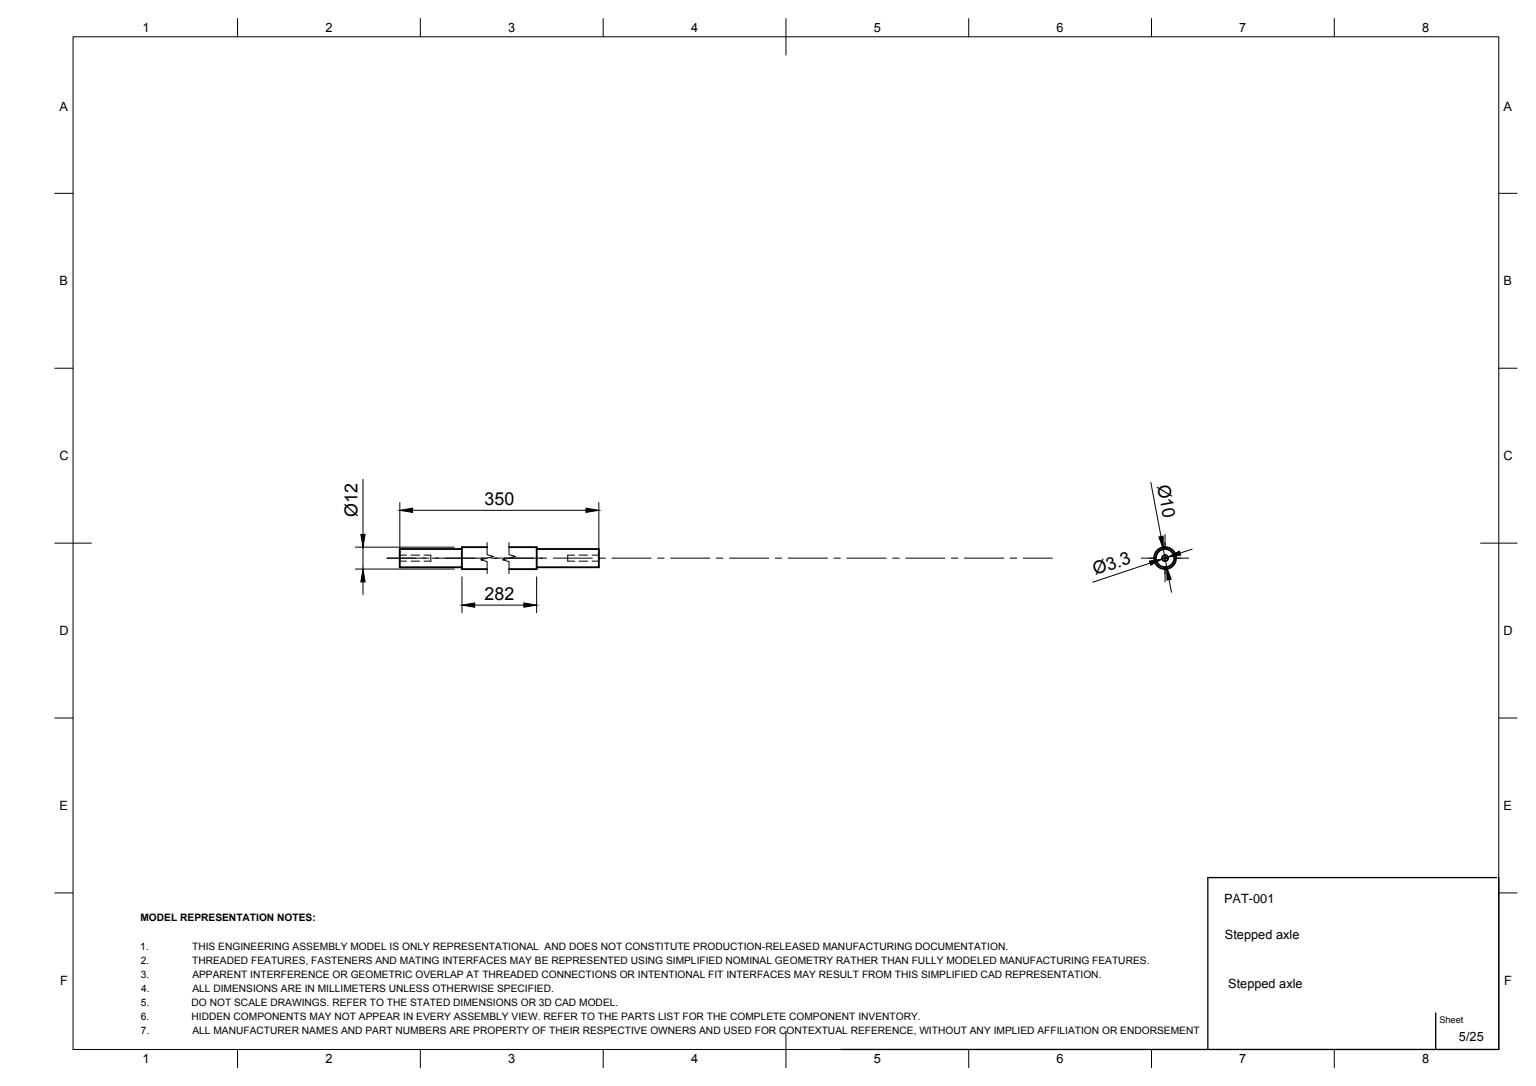
ISO-10303-21;
HEADER;
/* Generated by software containing ST-Developer
 * from STEP Tools, Inc. (www.steptools.com) 
 */

FILE_DESCRIPTION(
/* description */ ('PAT-001'),
/* implementation_level */ '2;1');

FILE_NAME(
/* name */ 'Stepped axle.step',
/* time_stamp */ '2026-10-29T17:07:15-07:00',
/* author */ (''),
/* organization */ (''),
/* preprocessor_version */ 'ST-DEVELOPER v20.2',
/* originating_system */ 'Autodesk Translation Framework v15.17.0.0',
/* authorisation */ '');

FILE_SCHEMA (('AUTOMOTIVE_DESIGN { 1 0 10303 214 3 1 1 }'));
ENDSEC;

DATA;
#10=MECHANICAL_DESIGN_GEOMETRIC_PRESENTATION_REPRESENTATION('',(#373),#9622);
#323=SHAPE_REPRESENTATION_RELATIONSHIP('SRR','None',#9746,#348);
#348=ADVANCED_BREP_SHAPE_REPRESENTATION('',(#406),#9595);
#373=STYLED_ITEM('',(#9962),#406);
#406=MANIFOLD_SOLID_BREP('Body1',#5198);
#437=FACE_BOUND('',#1016,.T.);
#438=FACE_BOUND('',#1018,.T.);
#439=FACE_BOUND('',#1023,.T.);
#440=FACE_BOUND('',#1025,.T.);
#528=PLANE('',#5515);
#529=PLANE('',#5519);
#530=PLANE('',#5520);
#531=PLANE('',#5523);
#532=PLANE('',#5531);
#533=PLANE('',#5532);
#715=FACE_OUTER_BOUND('',#1011,.T.);
#716=FACE_OUTER_BOUND('',#1012,.T.);
#717=FACE_OUTER_BOUND('',#1013,.T.);
#718=FACE_OUTER_BOUND('',#1014,.T.);
#719=FACE_OUTER_BOUND('',#1015,.T.);
#720=FACE_OUTER_BOUND('',#1017,.T.);
#721=FACE_OUTER_BOUND('',#1019,.T.);
#722=FACE_OUTER_BOUND('',#1020,.T.);
#723=FACE_OUTER_BOUND('',#1021,.T.);
#724=FACE_OUTER_BOUND('',#1022,.T.);
#725=FACE_OUTER_BOUND('',#1024,.T.);
#1011=EDGE_LOOP('',(#3517,#3518,#3519,#3520));
#1012=EDGE_LOOP('',(#3521));
#1013=EDGE_LOOP('',(#3522,#3523,#3524,#3525));
#1014=EDGE_LOOP('',(#3526));
#1015=EDGE_LOOP('',(#3527));
#1016=EDGE_LOOP('',(#3528));
#1017=EDGE_LOOP('',(#3529));
#1018=EDGE_LOOP('',(#3530));
#1019=EDGE_LOOP('',(#3531,#3532,#3533,#3534));
#1020=EDGE_LOOP('',(#3535,#3536,#3537,#3538));
#1021=EDGE_LOOP('',(#3539,#3540,#3541,#3542));
#1022=EDGE_LOOP('',(#3543));
#1023=EDGE_LOOP('',(#3544));
#1024=EDGE_LOOP('',(#3545));
#1025=EDGE_LOOP('',(#3546));
#1398=LINE('',#7715,#1803);
#1399=LINE('',#7722,#1804);
#1400=LINE('',#7736,#1805);
#1401=LINE('',#7739,#1806);
#1402=LINE('',#7744,#1807);
#1803=VECTOR('',#6117,0.165);
#1804=VECTOR('',#6126,0.165);
#1805=VECTOR('',#6145,0.6);
#1806=VECTOR('',#6148,0.5);
#1807=VECTOR('',#6155,0.5);
#2208=CIRCLE('',#5513,0.165);
#2209=CIRCLE('',#5514,0.165);
#2210=CIRCLE('',#5517,0.165);
#2211=CIRCLE('',#5518,0.165);
#2212=CIRCLE('',#5521,0.6);
#2213=CIRCLE('',#5522,0.5);
#2214=CIRCLE('',#5524,0.6);
#2215=CIRCLE('',#5525,0.5);
#2216=CIRCLE('',#5528,0.5);
#2217=CIRCLE('',#5530,0.5);
#2420=VERTEX_POINT('',#7712);
#2421=VERTEX_POINT('',#7714);
#2422=VERTEX_POINT('',#7719);
#2423=VERTEX_POINT('',#7721);
#2424=VERTEX_POINT('',#7726);
#2425=VERTEX_POINT('',#7728);
#2426=VERTEX_POINT('',#7731);
#2427=VERTEX_POINT('',#7733);
#2428=VERTEX_POINT('',#7738);
#2429=VERTEX_POINT('',#7742);
#2862=EDGE_CURVE('',#2420,#2420,#2208,.T.);
#2863=EDGE_CURVE('',#2420,#2421,#1398,.T.);
#2864=EDGE_CURVE('',#2421,#2421,#2209,.T.);
#2865=EDGE_CURVE('',#2422,#2422,#2210,.T.);
#2866=EDGE_CURVE('',#2422,#2423,#1399,.T.);
#2867=EDGE_CURVE('',#2423,#2423,#2211,.T.);
#2868=EDGE_CURVE('',#2424,#2424,#2212,.T.);
#2869=EDGE_CURVE('',#2425,#2425,#2213,.T.);
#2870=EDGE_CURVE('',#2426,#2426,#2214,.T.);
#2871=EDGE_CURVE('',#2427,#2427,#2215,.T.);
#2872=EDGE_CURVE('',#2424,#2426,#1400,.T.);
#2873=EDGE_CURVE('',#2427,#2428,#1401,.T.);
#2874=EDGE_CURVE('',#2428,#2428,#2216,.T.);
#2875=EDGE_CURVE('',#2429,#2429,#2217,.T.);
#2876=EDGE_CURVE('',#2429,#2425,#1402,.T.);
#3517=ORIENTED_EDGE('',*,*,#2862,.F.);
#3518=ORIENTED_EDGE('',*,*,#2863,.T.);
#3519=ORIENTED_EDGE('',*,*,#2864,.F.);
#3520=ORIENTED_EDGE('',*,*,#2863,.F.);
#3521=ORIENTED_EDGE('',*,*,#2862,.T.);
#3522=ORIENTED_EDGE('',*,*,#2865,.F.);
#3523=ORIENTED_EDGE('',*,*,#2866,.T.);
#3524=ORIENTED_EDGE('',*,*,#2867,.T.);
#3525=ORIENTED_EDGE('',*,*,#2866,.F.);
#3526=ORIENTED_EDGE('',*,*,#2867,.F.);
#3527=ORIENTED_EDGE('',*,*,#2868,.T.);
#3528=ORIENTED_EDGE('',*,*,#2869,.F.);
#3529=ORIENTED_EDGE('',*,*,#2870,.F.);
#3530=ORIENTED_EDGE('',*,*,#2871,.F.);
#3531=ORIENTED_EDGE('',*,*,#2868,.F.);
#3532=ORIENTED_EDGE('',*,*,#2872,.T.);
#3533=ORIENTED_EDGE('',*,*,#2870,.T.);
#3534=ORIENTED_EDGE('',*,*,#2872,.F.);
#3535=ORIENTED_EDGE('',*,*,#2871,.T.);
#3536=ORIENTED_EDGE('',*,*,#2873,.T.);
#3537=ORIENTED_EDGE('',*,*,#2874,.T.);
#3538=ORIENTED_EDGE('',*,*,#2873,.F.);
#3539=ORIENTED_EDGE('',*,*,#2875,.F.);
#3540=ORIENTED_EDGE('',*,*,#2876,.T.);
#3541=ORIENTED_EDGE('',*,*,#2869,.T.);
#3542=ORIENTED_EDGE('',*,*,#2876,.F.);
#3543=ORIENTED_EDGE('',*,*,#2875,.T.);
#3544=ORIENTED_EDGE('',*,*,#2864,.T.);
#3545=ORIENTED_EDGE('',*,*,#2874,.F.);
#3546=ORIENTED_EDGE('',*,*,#2865,.T.);
#4827=CYLINDRICAL_SURFACE('',#5512,0.165);
#4828=CYLINDRICAL_SURFACE('',#5516,0.165);
#4829=CYLINDRICAL_SURFACE('',#5526,0.6);
#4830=CYLINDRICAL_SURFACE('',#5527,0.5);
#4831=CYLINDRICAL_SURFACE('',#5529,0.5);
#4902=ADVANCED_FACE('',(#715),#4827,.F.);
#4903=ADVANCED_FACE('',(#716),#528,.T.);
#4904=ADVANCED_FACE('',(#717),#4828,.F.);
#4905=ADVANCED_FACE('',(#718),#529,.F.);
#4906=ADVANCED_FACE('',(#719,#437),#530,.T.);
#4907=ADVANCED_FACE('',(#720,#438),#531,.F.);
#4908=ADVANCED_FACE('',(#721),#4829,.T.);
#4909=ADVANCED_FACE('',(#722),#4830,.T.);
#4910=ADVANCED_FACE('',(#723),#4831,.T.);
#4911=ADVANCED_FACE('',(#724,#439),#532,.T.);
#4912=ADVANCED_FACE('',(#725,#440),#533,.F.);
#5198=CLOSED_SHELL('',(#4902,#4903,#4904,#4905,#4906,#4907,#4908,#4909,
#4910,#4911,#4912));
#5511=AXIS2_PLACEMENT_3D('',#7710,#6111,#6112);
#5512=AXIS2_PLACEMENT_3D('',#7711,#6113,#6114);
#5513=AXIS2_PLACEMENT_3D('',#7713,#6115,#6116);
#5514=AXIS2_PLACEMENT_3D('',#7716,#6118,#6119);
#5515=AXIS2_PLACEMENT_3D('',#7717,#6120,#6121);
#5516=AXIS2_PLACEMENT_3D('',#7718,#6122,#6123);
#5517=AXIS2_PLACEMENT_3D('',#7720,#6124,#6125);
#5518=AXIS2_PLACEMENT_3D('',#7723,#6127,#6128);
#5519=AXIS2_PLACEMENT_3D('',#7724,#6129,#6130);
#5520=AXIS2_PLACEMENT_3D('',#7725,#6131,#6132);
#5521=AXIS2_PLACEMENT_3D('',#7727,#6133,#6134);
#5522=AXIS2_PLACEMENT_3D('',#7729,#6135,#6136);
#5523=AXIS2_PLACEMENT_3D('',#7730,#6137,#6138);
#5524=AXIS2_PLACEMENT_3D('',#7732,#6139,#6140);
#5525=AXIS2_PLACEMENT_3D('',#7734,#6141,#6142);
#5526=AXIS2_PLACEMENT_3D('',#7735,#6143,#6144);
#5527=AXIS2_PLACEMENT_3D('',#7737,#6146,#6147);
#5528=AXIS2_PLACEMENT_3D('',#7740,#6149,#6150);
#5529=AXIS2_PLACEMENT_3D('',#7741,#6151,#6152);
#5530=AXIS2_PLACEMENT_3D('',#7743,#6153,#6154);
#5531=AXIS2_PLACEMENT_3D('',#7745,#6156,#6157);
#5532=AXIS2_PLACEMENT_3D('',#7746,#6158,#6159);
#6111=DIRECTION('axis',(0.,0.,1.));
#6112=DIRECTION('refdir',(1.,0.,0.));
#6113=DIRECTION('center_axis',(0.,1.,0.));
#6114=DIRECTION('ref_axis',(1.,0.,0.));
#6115=DIRECTION('center_axis',(0.,1.,0.));
#6116=DIRECTION('ref_axis',(1.,0.,0.));
#6117=DIRECTION('',(0.,1.,0.));
#6118=DIRECTION('center_axis',(0.,-1.,0.));
#6119=DIRECTION('ref_axis',(1.,0.,0.));
#6120=DIRECTION('center_axis',(0.,1.,0.));
#6121=DIRECTION('ref_axis',(1.,0.,0.));
#6122=DIRECTION('center_axis',(0.,1.,0.));
#6123=DIRECTION('ref_axis',(1.,0.,0.));
#6124=DIRECTION('center_axis',(0.,1.,0.));
#6125=DIRECTION('ref_axis',(1.,0.,0.));
#6126=DIRECTION('',(0.,1.,0.));
#6127=DIRECTION('center_axis',(0.,1.,0.));
#6128=DIRECTION('ref_axis',(1.,0.,0.));
#6129=DIRECTION('center_axis',(0.,1.,0.));
#6130=DIRECTION('ref_axis',(1.,0.,0.));
#6131=DIRECTION('center_axis',(0.,1.,0.));
#6132=DIRECTION('ref_axis',(1.,0.,0.));
#6133=DIRECTION('center_axis',(0.,1.,0.));
#6134=DIRECTION('ref_axis',(1.,0.,0.));
#6135=DIRECTION('center_axis',(0.,1.,0.));
#6136=DIRECTION('ref_axis',(1.,0.,0.));
#6137=DIRECTION('center_axis',(0.,1.,0.));
#6138=DIRECTION('ref_axis',(1.,0.,0.));
#6139=DIRECTION('center_axis',(0.,1.,0.));
#6140=DIRECTION('ref_axis',(1.,0.,0.));
#6141=DIRECTION('center_axis',(0.,-1.,0.));
#6142=DIRECTION('ref_axis',(1.,0.,0.));
#6143=DIRECTION('center_axis',(0.,1.,0.));
#6144=DIRECTION('ref_axis',(1.,0.,0.));
#6145=DIRECTION('',(0.,-1.,0.));
#6146=DIRECTION('center_axis',(0.,1.,0.));
#6147=DIRECTION('ref_axis',(1.,0.,0.));
#6148=DIRECTION('',(0.,-1.,0.));
#6149=DIRECTION('center_axis',(0.,1.,0.));
#6150=DIRECTION('ref_axis',(1.,0.,0.));
#6151=DIRECTION('center_axis',(0.,1.,0.));
#6152=DIRECTION('ref_axis',(1.,0.,0.));
#6153=DIRECTION('center_axis',(0.,1.,0.));
#6154=DIRECTION('ref_axis',(1.,0.,0.));
#6155=DIRECTION('',(0.,-1.,0.));
#6156=DIRECTION('center_axis',(0.,1.,0.));
#6157=DIRECTION('ref_axis',(1.,0.,0.));
#6158=DIRECTION('center_axis',(0.,1.,0.));
#6159=DIRECTION('ref_axis',(1.,0.,0.));
#7710=CARTESIAN_POINT('',(0.,0.,0.));
#7711=CARTESIAN_POINT('Origin',(0.,30.8,4.5));
#7712=CARTESIAN_POINT('',(-0.165,30.8,4.5));
#7713=CARTESIAN_POINT('Origin',(0.,30.8,4.5));
#7714=CARTESIAN_POINT('',(-0.165,32.5,4.5));
#7715=CARTESIAN_POINT('',(-0.165,30.8,4.5));
#7716=CARTESIAN_POINT('Origin',(0.,32.5,4.5));
#7717=CARTESIAN_POINT('Origin',(0.,30.8,4.5));
#7718=CARTESIAN_POINT('Origin',(0.,-2.6,4.5));
#7719=CARTESIAN_POINT('',(-0.165,-2.5,4.5));
#7720=CARTESIAN_POINT('Origin',(0.,-2.5,4.5));
#7721=CARTESIAN_POINT('',(-0.165,-0.8,4.5));
#7722=CARTESIAN_POINT('',(-0.165,-2.6,4.5));
#7723=CARTESIAN_POINT('Origin',(0.,-0.8,4.5));
#7724=CARTESIAN_POINT('Origin',(0.,-0.8,4.5));
#7725=CARTESIAN_POINT('Origin',(0.,29.1,4.5));
#7726=CARTESIAN_POINT('',(-0.6,29.1,4.5));
#7727=CARTESIAN_POINT('Origin',(0.,29.1,4.5));
#7728=CARTESIAN_POINT('',(-0.5,29.1,4.5));
#7729=CARTESIAN_POINT('Origin',(0.,29.1,4.5));
#7730=CARTESIAN_POINT('Origin',(0.,0.9,4.5));
#7731=CARTESIAN_POINT('',(-0.6,0.9,4.5));
#7732=CARTESIAN_POINT('Origin',(0.,0.9,4.5));
#7733=CARTESIAN_POINT('',(-0.5,0.9,4.5));
#7734=CARTESIAN_POINT('Origin',(0.,0.9,4.5));
#7735=CARTESIAN_POINT('Origin',(0.,0.9,4.5));
#7736=CARTESIAN_POINT('',(-0.6,0.9,4.5));
#7737=CARTESIAN_POINT('Origin',(0.,-2.5,4.5));
#7738=CARTESIAN_POINT('',(-0.5,-2.5,4.5));
#7739=CARTESIAN_POINT('',(-0.5,-2.5,4.5));
#7740=CARTESIAN_POINT('Origin',(0.,-2.5,4.5));
#7741=CARTESIAN_POINT('Origin',(0.,-2.5,4.5));
#7742=CARTESIAN_POINT('',(-0.5,32.5,4.5));
#7743=CARTESIAN_POINT('Origin',(0.,32.5,4.5));
#7744=CARTESIAN_POINT('',(-0.5,-2.5,4.5));
#7745=CARTESIAN_POINT('Origin',(0.,32.5,4.5));
#7746=CARTESIAN_POINT('Origin',(0.,-2.5,4.5));
#9565=UNCERTAINTY_MEASURE_WITH_UNIT(LENGTH_MEASURE(0.001),#9623,
'DISTANCE_ACCURACY_VALUE',
'Maximum model space distance between geometric entities at asserted c
onnectivities');
#9592=UNCERTAINTY_MEASURE_WITH_UNIT(LENGTH_MEASURE(0.001),#9623,
'DISTANCE_ACCURACY_VALUE',
'Maximum model space distance between geometric entities at asserted c
onnectivities');
#9595=(
GEOMETRIC_REPRESENTATION_CONTEXT(3)
GLOBAL_UNCERTAINTY_ASSIGNED_CONTEXT((#9565))
GLOBAL_UNIT_ASSIGNED_CONTEXT((#9623,#9625,#9626))
REPRESENTATION_CONTEXT('','3D')
);
#9622=(
GEOMETRIC_REPRESENTATION_CONTEXT(3)
GLOBAL_UNCERTAINTY_ASSIGNED_CONTEXT((#9592))
GLOBAL_UNIT_ASSIGNED_CONTEXT((#9623,#9625,#9626))
REPRESENTATION_CONTEXT('','3D')
);
#9623=(
LENGTH_UNIT()
NAMED_UNIT(*)
SI_UNIT(.CENTI.,.METRE.)
);
#9625=(
NAMED_UNIT(*)
PLANE_ANGLE_UNIT()
SI_UNIT($,.RADIAN.)
);
#9626=(
NAMED_UNIT(*)
SI_UNIT($,.STERADIAN.)
SOLID_ANGLE_UNIT()
);
#9629=SHAPE_DEFINITION_REPRESENTATION(#9658,#9746);
#9658=PRODUCT_DEFINITION_SHAPE('',$,#9776);
#9746=SHAPE_REPRESENTATION('',(#5511),#9595);
#9773=PRODUCT_DEFINITION_CONTEXT('part definition',#9862,'design');
#9776=PRODUCT_DEFINITION('Stepped axle','Stepped axle',#9805,#9773);
#9805=PRODUCT_DEFINITION_FORMATION('',$,#9866);
#9862=APPLICATION_CONTEXT(
'Core Data for Automotive Mechanical Design Process');
#9863=PRODUCT_CONTEXT('part definition',#9862,'mechanical');
#9866=PRODUCT('Stepped axle','Stepped axle','Stepped axle',(#9863));
#9956=COLOUR_RGB('Grey',0.48,0.52,0.57);
#9957=FILL_AREA_STYLE_COLOUR('',#9956);
#9958=FILL_AREA_STYLE('',(#9957));
#9959=SURFACE_STYLE_FILL_AREA(#9958);
#9960=SURFACE_SIDE_STYLE('',(#9959));
#9961=SURFACE_STYLE_USAGE(.BOTH.,#9960);
#9962=PRESENTATION_STYLE_ASSIGNMENT((#9961));
ENDSEC;
END-ISO-10303-21;
